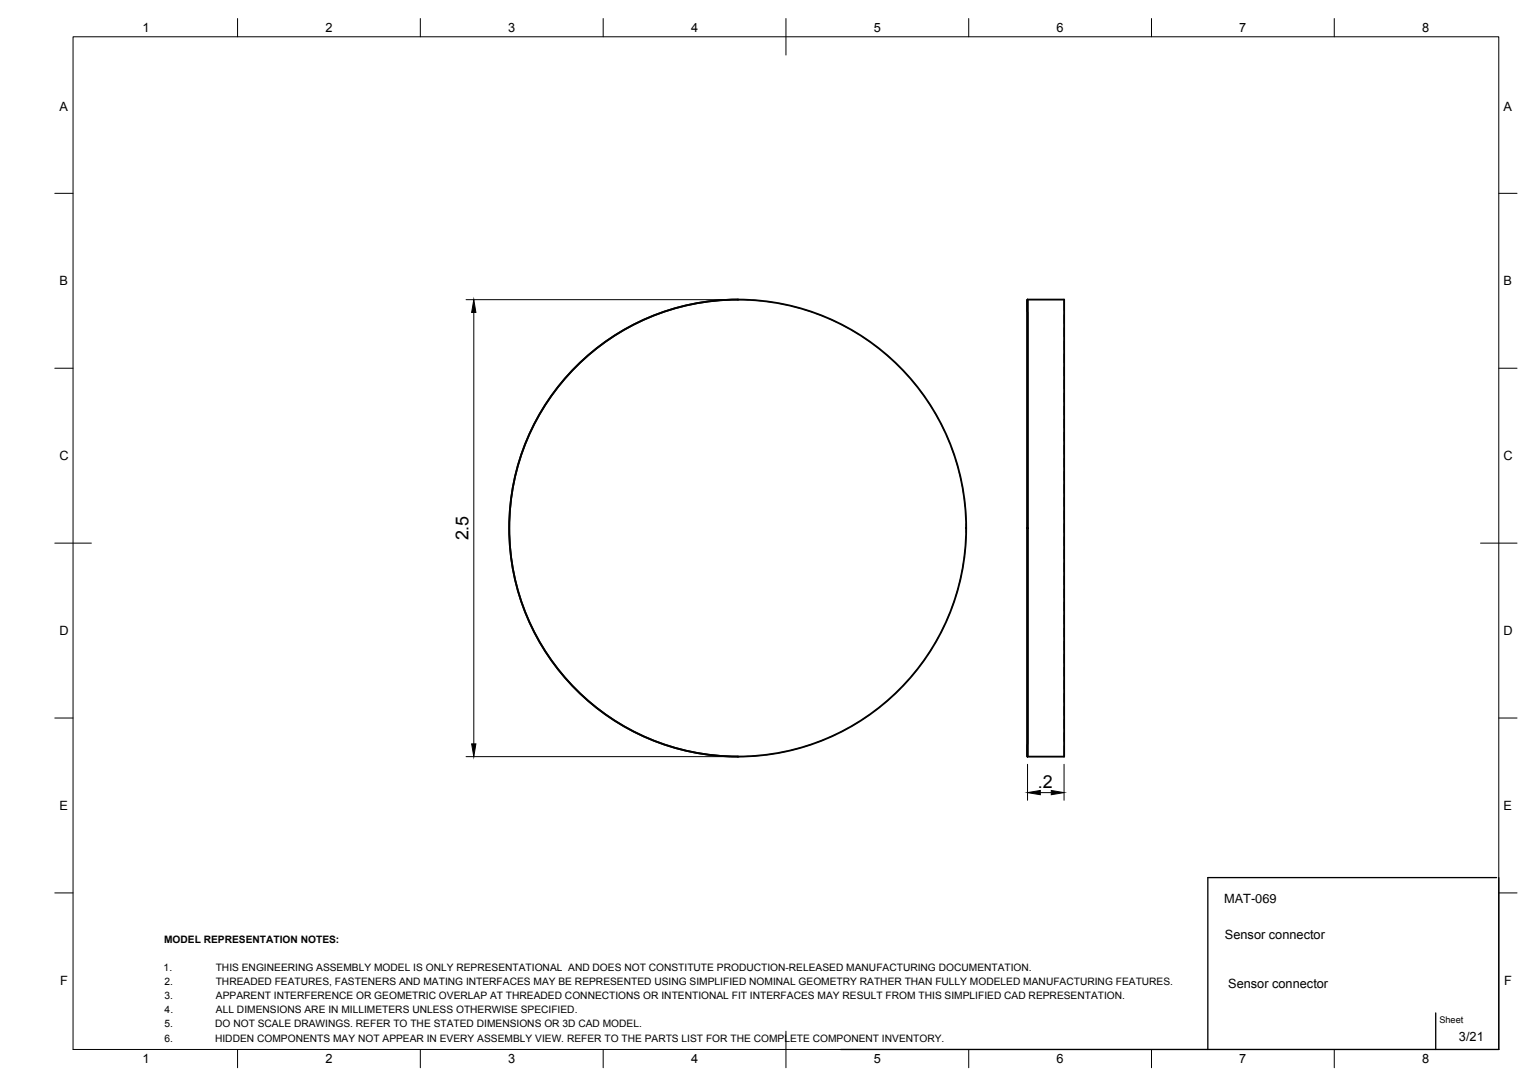
ISO-10303-21;
HEADER;
/* Generated by software containing ST-Developer
 * from STEP Tools, Inc. (www.steptools.com) 
 */

FILE_DESCRIPTION(
/* description */ ('CAx-IF Rec.Pracs.---Representation and Presentation of Product Manufa
cturing Information (PMI)---4.0---2014-10-13'),
/* implementation_level */ '2;1');

FILE_NAME(
/* name */ 'Sensor connector.step',
/* time_stamp */ '2026-10-24T15:08:39-07:00',
/* author */ (''),
/* organization */ (''),
/* preprocessor_version */ 'ST-DEVELOPER v20.2',
/* originating_system */ 'Autodesk Translation Framework v15.17.0.0',
/* authorisation */ '');

FILE_SCHEMA (('AP242_MANAGED_MODEL_BASED_3D_ENGINEERING_MIM_LF { 1 0 10303 442 2 1 4 }'));
ENDSEC;

DATA;
#10=MECHANICAL_DESIGN_GEOMETRIC_PRESENTATION_REPRESENTATION('',(#820),#50081);
#780=SHAPE_REPRESENTATION_RELATIONSHIP('SRR','None',#50148,#800);
#800=ADVANCED_BREP_SHAPE_REPRESENTATION('',(#840),#50061);
#820=STYLED_ITEM('',(#50257),#840);
#840=MANIFOLD_SOLID_BREP('Body1',#9865);
#860=PLANE('',#10111);
#861=PLANE('',#10112);
#1102=FACE_OUTER_BOUND('',#1643,.T.);
#1103=FACE_OUTER_BOUND('',#1644,.T.);
#1104=FACE_OUTER_BOUND('',#1645,.T.);
#1643=EDGE_LOOP('',(#6226,#6227,#6228,#6229));
#1644=EDGE_LOOP('',(#6230));
#1645=EDGE_LOOP('',(#6231));
#2243=LINE('',#13477,#2821);
#2821=VECTOR('',#11043,0.00125);
#3399=CIRCLE('',#10109,0.00125000000001);
#3400=CIRCLE('',#10110,0.00125000000001);
#3772=VERTEX_POINT('',#13474);
#3773=VERTEX_POINT('',#13476);
#4766=EDGE_CURVE('',#3772,#3772,#3399,.T.);
#4767=EDGE_CURVE('',#3772,#3773,#2243,.T.);
#4768=EDGE_CURVE('',#3773,#3773,#3400,.T.);
#6226=ORIENTED_EDGE('',*,*,#4766,.F.);
#6227=ORIENTED_EDGE('',*,*,#4767,.T.);
#6228=ORIENTED_EDGE('',*,*,#4768,.T.);
#6229=ORIENTED_EDGE('',*,*,#4767,.F.);
#6230=ORIENTED_EDGE('',*,*,#4766,.T.);
#6231=ORIENTED_EDGE('',*,*,#4768,.F.);
#9146=CYLINDRICAL_SURFACE('',#10108,0.00125);
#9324=ADVANCED_FACE('',(#1102),#9146,.T.);
#9325=ADVANCED_FACE('',(#1103),#860,.T.);
#9326=ADVANCED_FACE('',(#1104),#861,.F.);
#9865=CLOSED_SHELL('',(#9324,#9325,#9326));
#10107=AXIS2_PLACEMENT_3D('',#13472,#11037,#11038);
#10108=AXIS2_PLACEMENT_3D('',#13473,#11039,#11040);
#10109=AXIS2_PLACEMENT_3D('',#13475,#11041,#11042);
#10110=AXIS2_PLACEMENT_3D('',#13478,#11044,#11045);
#10111=AXIS2_PLACEMENT_3D('',#13479,#11046,#11047);
#10112=AXIS2_PLACEMENT_3D('',#13480,#11048,#11049);
#11037=DIRECTION('axis',(0.,0.,1.));
#11038=DIRECTION('refdir',(1.,0.,0.));
#11039=DIRECTION('center_axis',(-2.42833204006769E-16,-2.41473507855972E-15,
1.));
#11040=DIRECTION('ref_axis',(-0.422618261740706,-0.906307787036647,-2.29111895189949E-15));
#11041=DIRECTION('center_axis',(-2.42833204006769E-16,-2.41473507855972E-15,
1.));
#11042=DIRECTION('ref_axis',(-0.422618261740706,-0.906307787036647,-2.29111895189949E-15));
#11043=DIRECTION('',(2.42833204006769E-16,2.41473507855972E-15,-1.));
#11044=DIRECTION('center_axis',(-2.42833204006769E-16,-2.41473507855972E-15,
1.));
#11045=DIRECTION('ref_axis',(-0.422618261740706,-0.906307787036647,-2.29111895189949E-15));
#11046=DIRECTION('center_axis',(-2.42833204006769E-16,-2.41473507855972E-15,
1.));
#11047=DIRECTION('ref_axis',(0.422618261740706,0.906307787036647,2.29111895189949E-15));
#11048=DIRECTION('center_axis',(-2.42833204006769E-16,-2.41473507855972E-15,
1.));
#11049=DIRECTION('ref_axis',(0.422618261740706,0.906307787036647,2.29111895189949E-15));
#13472=CARTESIAN_POINT('',(0.,0.,0.));
#13473=CARTESIAN_POINT('Origin',(0.006,-0.0355287743898724,-0.0045758532865581));
#13474=CARTESIAN_POINT('',(0.00652827282717588,-0.0343958896560766,-0.0043758532865481));
#13475=CARTESIAN_POINT('Origin',(0.006,-0.0355287743898724,-0.0043758532865481));
#13476=CARTESIAN_POINT('',(0.00652827282717588,-0.0343958896560766,-0.0045758532865481));
#13477=CARTESIAN_POINT('',(0.00652827282717588,-0.0343958896560766,-0.0045758532865581));
#13478=CARTESIAN_POINT('Origin',(0.006,-0.0355287743898724,-0.0045758532865481));
#13479=CARTESIAN_POINT('Origin',(0.006,-0.0355287743898724,-0.0043758532865581));
#13480=CARTESIAN_POINT('Origin',(0.006,-0.0355287743898724,-0.0045758532865581));
#50039=UNCERTAINTY_MEASURE_WITH_UNIT(LENGTH_MEASURE(1.E-5),#50082,
'DISTANCE_ACCURACY_VALUE',
'Maximum model space distance between geometric entities at asserted c
onnectivities');
#50059=UNCERTAINTY_MEASURE_WITH_UNIT(LENGTH_MEASURE(1.E-5),#50082,
'DISTANCE_ACCURACY_VALUE',
'Maximum model space distance between geometric entities at asserted c
onnectivities');
#50061=(
GEOMETRIC_REPRESENTATION_CONTEXT(3)
GLOBAL_UNCERTAINTY_ASSIGNED_CONTEXT((#50039))
GLOBAL_UNIT_ASSIGNED_CONTEXT((#50082,#50083,#50084))
REPRESENTATION_CONTEXT('','3D')
);
#50081=(
GEOMETRIC_REPRESENTATION_CONTEXT(3)
GLOBAL_UNCERTAINTY_ASSIGNED_CONTEXT((#50059))
GLOBAL_UNIT_ASSIGNED_CONTEXT((#50082,#50083,#50084))
REPRESENTATION_CONTEXT('','3D')
);
#50082=(
LENGTH_UNIT()
NAMED_UNIT(*)
SI_UNIT($,.METRE.)
);
#50083=(
NAMED_UNIT(*)
PLANE_ANGLE_UNIT()
SI_UNIT($,.RADIAN.)
);
#50084=(
NAMED_UNIT(*)
SI_UNIT($,.STERADIAN.)
SOLID_ANGLE_UNIT()
);
#50086=SHAPE_DEFINITION_REPRESENTATION(#50107,#50148);
#50107=PRODUCT_DEFINITION_SHAPE('',$,#50170);
#50148=SHAPE_REPRESENTATION('',(#10107),#50061);
#50168=PRODUCT_DEFINITION_CONTEXT('part definition',#50233,'design');
#50170=PRODUCT_DEFINITION('Sensor connector','Sensor connector',#50191,
#50168);
#50191=PRODUCT_DEFINITION_FORMATION('',$,#50236);
#50233=APPLICATION_CONTEXT('Managed model based 3d engineering');
#50234=PRODUCT_CONTEXT('part definition',#50233,'mechanical');
#50236=PRODUCT('Sensor connector','Sensor connector',
'LEGAL AND USAGE DISCLAIMER: this Data/Model is provided \X2\201C\X0\A
S IS\X2\201D\X0\ for informational and representational only. It is a 
geometric approximation and is NOT engineered, certified, or guarantee
d for dimensional accuracy, exact tolerances, or production-level prec
ision. Vendor disclaims all implied warranties including fitness for a
 particular purpose. DO NOT USE FOR DIRECT PHYSICAL MANUFACTURING, AUT
OMATED PRODUCTION, OR SAFETY-CRITICAL SYSTEMS without independent engi
neering verification and resolution of any design discrepancies.',(#50234));
#50257=PRESENTATION_STYLE_ASSIGNMENT((#50264));
#50264=SURFACE_STYLE_USAGE(.BOTH.,#50271);
#50271=SURFACE_SIDE_STYLE('',(#50278));
#50278=SURFACE_STYLE_FILL_AREA(#50285);
#50285=FILL_AREA_STYLE('Opaque(137,137,137)',(#50292));
#50292=FILL_AREA_STYLE_COLOUR('Opaque(137,137,137)',#50299);
#50299=COLOUR_RGB('Opaque(137,137,137)',0.537254901960784,0.537254901960784,
0.537254901960784);
ENDSEC;
END-ISO-10303-21;
